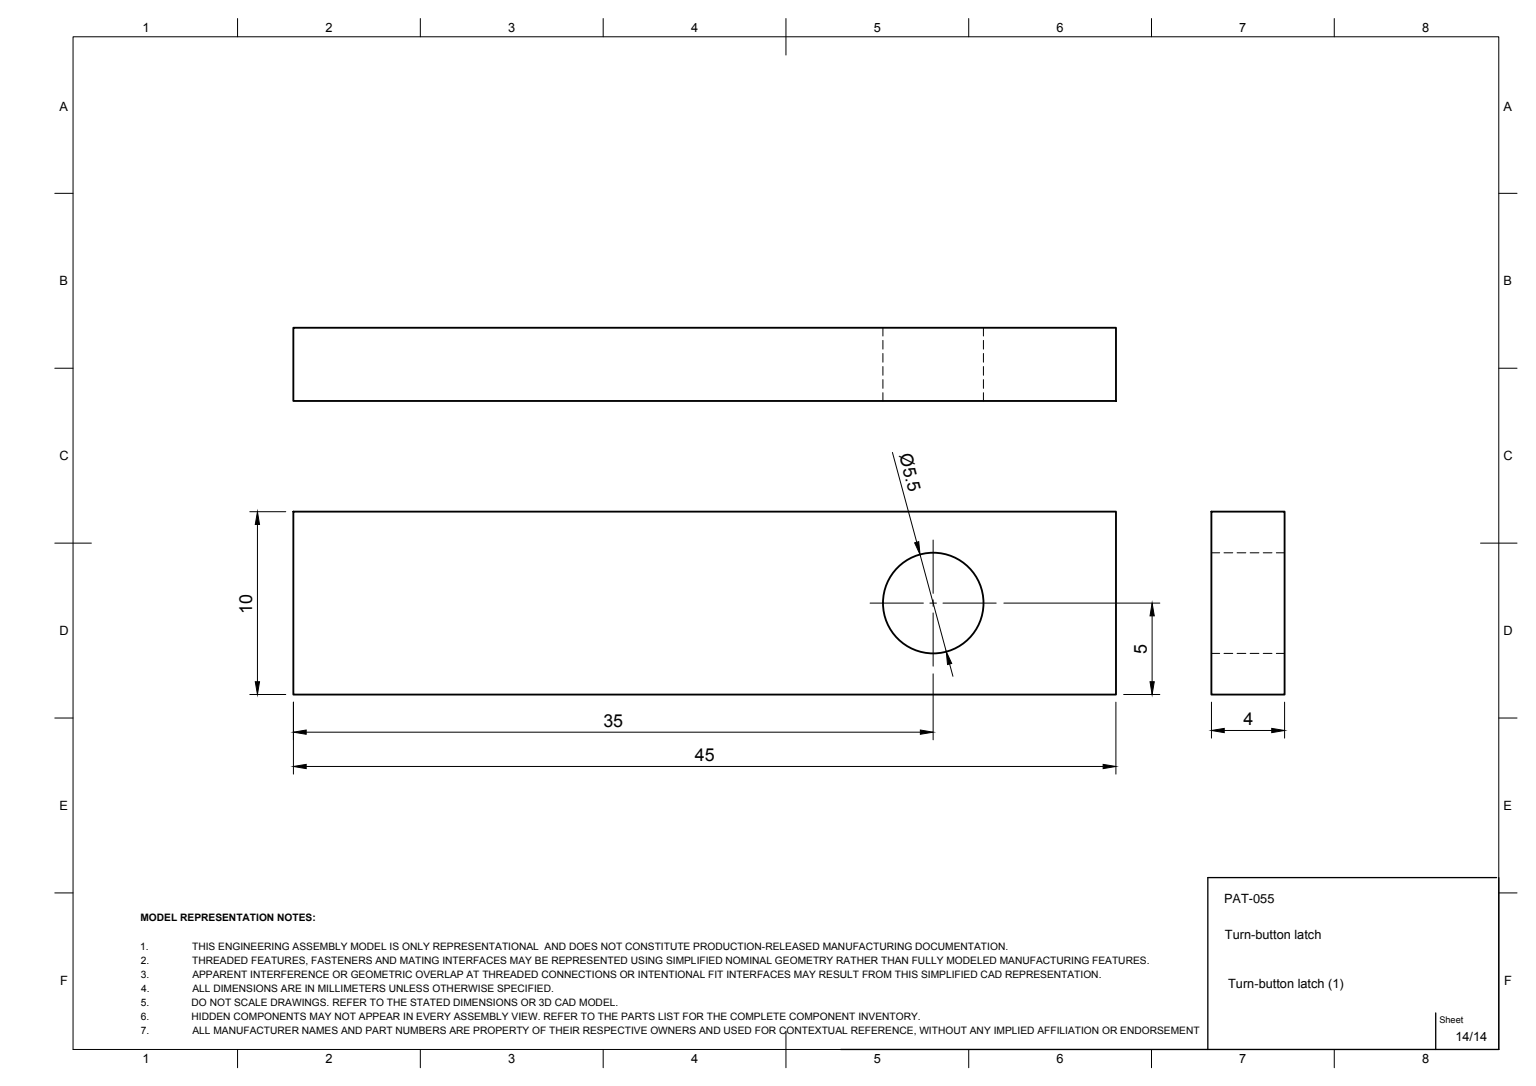
ISO-10303-21;
HEADER;
/* Generated by software containing ST-Developer
 * from STEP Tools, Inc. (www.steptools.com) 
 */

FILE_DESCRIPTION(
/* description */ ('Hinged panel with latch'),
/* implementation_level */ '2;1');

FILE_NAME(
/* name */ 'Turn-button latch (1).step',
/* time_stamp */ '2026-10-27T20:36:01-07:00',
/* author */ (''),
/* organization */ (''),
/* preprocessor_version */ 'ST-DEVELOPER v20.2',
/* originating_system */ 'Autodesk Translation Framework v15.17.0.0',
/* authorisation */ '');

FILE_SCHEMA (('AUTOMOTIVE_DESIGN { 1 0 10303 214 3 1 1 }'));
ENDSEC;

DATA;
#10=MECHANICAL_DESIGN_GEOMETRIC_PRESENTATION_REPRESENTATION('',(#311),#6743);
#279=SHAPE_REPRESENTATION_RELATIONSHIP('SRR','None',#6856,#295);
#295=ADVANCED_BREP_SHAPE_REPRESENTATION('',(#324),#6742);
#311=STYLED_ITEM('',(#6989),#324);
#324=MANIFOLD_SOLID_BREP('Body1',#3816);
#370=FACE_BOUND('',#975,.T.);
#371=FACE_BOUND('',#978,.T.);
#517=PLANE('',#4354);
#518=PLANE('',#4355);
#519=PLANE('',#4356);
#520=PLANE('',#4357);
#521=PLANE('',#4358);
#522=PLANE('',#4359);
#722=FACE_OUTER_BOUND('',#973,.T.);
#723=FACE_OUTER_BOUND('',#974,.T.);
#724=FACE_OUTER_BOUND('',#976,.T.);
#725=FACE_OUTER_BOUND('',#977,.T.);
#726=FACE_OUTER_BOUND('',#979,.T.);
#727=FACE_OUTER_BOUND('',#980,.T.);
#728=FACE_OUTER_BOUND('',#981,.T.);
#973=EDGE_LOOP('',(#3526,#3527,#3528,#3529));
#974=EDGE_LOOP('',(#3530,#3531,#3532,#3533));
#975=EDGE_LOOP('',(#3534));
#976=EDGE_LOOP('',(#3535,#3536,#3537,#3538));
#977=EDGE_LOOP('',(#3539,#3540,#3541,#3542));
#978=EDGE_LOOP('',(#3543));
#979=EDGE_LOOP('',(#3544,#3545,#3546,#3547));
#980=EDGE_LOOP('',(#3548,#3549,#3550,#3551));
#981=EDGE_LOOP('',(#3552,#3553,#3554,#3555));
#1327=LINE('',#6670,#1685);
#1328=LINE('',#6675,#1686);
#1329=LINE('',#6677,#1687);
#1330=LINE('',#6679,#1688);
#1331=LINE('',#6680,#1689);
#1332=LINE('',#6683,#1690);
#1333=LINE('',#6685,#1691);
#1334=LINE('',#6686,#1692);
#1335=LINE('',#6689,#1693);
#1336=LINE('',#6691,#1694);
#1337=LINE('',#6692,#1695);
#1338=LINE('',#6694,#1696);
#1339=LINE('',#6695,#1697);
#1685=VECTOR('',#5427,0.274999999999999);
#1686=VECTOR('',#5432,1.);
#1687=VECTOR('',#5433,1.);
#1688=VECTOR('',#5434,1.);
#1689=VECTOR('',#5435,1.);
#1690=VECTOR('',#5438,1.);
#1691=VECTOR('',#5439,1.);
#1692=VECTOR('',#5440,1.);
#1693=VECTOR('',#5443,1.);
#1694=VECTOR('',#5444,1.);
#1695=VECTOR('',#5445,1.);
#1696=VECTOR('',#5448,1.);
#1697=VECTOR('',#5449,1.);
#1789=CIRCLE('',#4352,0.274999999999999);
#1790=CIRCLE('',#4353,0.274999999999999);
#2097=VERTEX_POINT('',#6667);
#2098=VERTEX_POINT('',#6669);
#2099=VERTEX_POINT('',#6673);
#2100=VERTEX_POINT('',#6674);
#2101=VERTEX_POINT('',#6676);
#2102=VERTEX_POINT('',#6678);
#2103=VERTEX_POINT('',#6682);
#2104=VERTEX_POINT('',#6684);
#2105=VERTEX_POINT('',#6688);
#2106=VERTEX_POINT('',#6690);
#2575=EDGE_CURVE('',#2097,#2097,#1789,.T.);
#2576=EDGE_CURVE('',#2097,#2098,#1327,.T.);
#2577=EDGE_CURVE('',#2098,#2098,#1790,.T.);
#2578=EDGE_CURVE('',#2099,#2100,#1328,.T.);
#2579=EDGE_CURVE('',#2100,#2101,#1329,.T.);
#2580=EDGE_CURVE('',#2102,#2101,#1330,.T.);
#2581=EDGE_CURVE('',#2099,#2102,#1331,.T.);
#2582=EDGE_CURVE('',#2103,#2099,#1332,.T.);
#2583=EDGE_CURVE('',#2104,#2102,#1333,.T.);
#2584=EDGE_CURVE('',#2103,#2104,#1334,.T.);
#2585=EDGE_CURVE('',#2105,#2103,#1335,.T.);
#2586=EDGE_CURVE('',#2106,#2104,#1336,.T.);
#2587=EDGE_CURVE('',#2105,#2106,#1337,.T.);
#2588=EDGE_CURVE('',#2100,#2105,#1338,.T.);
#2589=EDGE_CURVE('',#2101,#2106,#1339,.T.);
#3526=ORIENTED_EDGE('',*,*,#2575,.F.);
#3527=ORIENTED_EDGE('',*,*,#2576,.T.);
#3528=ORIENTED_EDGE('',*,*,#2577,.F.);
#3529=ORIENTED_EDGE('',*,*,#2576,.F.);
#3530=ORIENTED_EDGE('',*,*,#2578,.T.);
#3531=ORIENTED_EDGE('',*,*,#2579,.T.);
#3532=ORIENTED_EDGE('',*,*,#2580,.F.);
#3533=ORIENTED_EDGE('',*,*,#2581,.F.);
#3534=ORIENTED_EDGE('',*,*,#2577,.T.);
#3535=ORIENTED_EDGE('',*,*,#2582,.T.);
#3536=ORIENTED_EDGE('',*,*,#2581,.T.);
#3537=ORIENTED_EDGE('',*,*,#2583,.F.);
#3538=ORIENTED_EDGE('',*,*,#2584,.F.);
#3539=ORIENTED_EDGE('',*,*,#2585,.T.);
#3540=ORIENTED_EDGE('',*,*,#2584,.T.);
#3541=ORIENTED_EDGE('',*,*,#2586,.F.);
#3542=ORIENTED_EDGE('',*,*,#2587,.F.);
#3543=ORIENTED_EDGE('',*,*,#2575,.T.);
#3544=ORIENTED_EDGE('',*,*,#2588,.T.);
#3545=ORIENTED_EDGE('',*,*,#2587,.T.);
#3546=ORIENTED_EDGE('',*,*,#2589,.F.);
#3547=ORIENTED_EDGE('',*,*,#2579,.F.);
#3548=ORIENTED_EDGE('',*,*,#2589,.T.);
#3549=ORIENTED_EDGE('',*,*,#2586,.T.);
#3550=ORIENTED_EDGE('',*,*,#2583,.T.);
#3551=ORIENTED_EDGE('',*,*,#2580,.T.);
#3552=ORIENTED_EDGE('',*,*,#2588,.F.);
#3553=ORIENTED_EDGE('',*,*,#2578,.F.);
#3554=ORIENTED_EDGE('',*,*,#2582,.F.);
#3555=ORIENTED_EDGE('',*,*,#2585,.F.);
#3591=CYLINDRICAL_SURFACE('',#4351,0.274999999999999);
#3791=ADVANCED_FACE('',(#722),#3591,.F.);
#3792=ADVANCED_FACE('',(#723,#370),#517,.T.);
#3793=ADVANCED_FACE('',(#724),#518,.T.);
#3794=ADVANCED_FACE('',(#725,#371),#519,.T.);
#3795=ADVANCED_FACE('',(#726),#520,.T.);
#3796=ADVANCED_FACE('',(#727),#521,.T.);
#3797=ADVANCED_FACE('',(#728),#522,.F.);
#3816=CLOSED_SHELL('',(#3791,#3792,#3793,#3794,#3795,#3796,#3797));
#4350=AXIS2_PLACEMENT_3D('',#6665,#5421,#5422);
#4351=AXIS2_PLACEMENT_3D('',#6666,#5423,#5424);
#4352=AXIS2_PLACEMENT_3D('',#6668,#5425,#5426);
#4353=AXIS2_PLACEMENT_3D('',#6671,#5428,#5429);
#4354=AXIS2_PLACEMENT_3D('',#6672,#5430,#5431);
#4355=AXIS2_PLACEMENT_3D('',#6681,#5436,#5437);
#4356=AXIS2_PLACEMENT_3D('',#6687,#5441,#5442);
#4357=AXIS2_PLACEMENT_3D('',#6693,#5446,#5447);
#4358=AXIS2_PLACEMENT_3D('',#6696,#5450,#5451);
#4359=AXIS2_PLACEMENT_3D('',#6697,#5452,#5453);
#5421=DIRECTION('axis',(0.,0.,1.));
#5422=DIRECTION('refdir',(1.,0.,0.));
#5423=DIRECTION('center_axis',(0.,1.,0.));
#5424=DIRECTION('ref_axis',(1.,0.,0.));
#5425=DIRECTION('center_axis',(0.,1.,0.));
#5426=DIRECTION('ref_axis',(1.,0.,0.));
#5427=DIRECTION('',(0.,1.,0.));
#5428=DIRECTION('center_axis',(0.,-1.,0.));
#5429=DIRECTION('ref_axis',(1.,0.,0.));
#5430=DIRECTION('center_axis',(0.,1.,0.));
#5431=DIRECTION('ref_axis',(-1.,0.,0.));
#5432=DIRECTION('',(-1.,0.,0.));
#5433=DIRECTION('',(0.,0.,1.));
#5434=DIRECTION('',(-1.,0.,0.));
#5435=DIRECTION('',(0.,0.,1.));
#5436=DIRECTION('center_axis',(1.,0.,0.));
#5437=DIRECTION('ref_axis',(0.,1.,0.));
#5438=DIRECTION('',(0.,1.,0.));
#5439=DIRECTION('',(0.,1.,0.));
#5440=DIRECTION('',(0.,0.,1.));
#5441=DIRECTION('center_axis',(0.,-1.,0.));
#5442=DIRECTION('ref_axis',(1.,0.,0.));
#5443=DIRECTION('',(1.,0.,0.));
#5444=DIRECTION('',(1.,0.,0.));
#5445=DIRECTION('',(0.,0.,1.));
#5446=DIRECTION('center_axis',(-1.,0.,0.));
#5447=DIRECTION('ref_axis',(0.,-1.,0.));
#5448=DIRECTION('',(0.,-1.,0.));
#5449=DIRECTION('',(0.,-1.,0.));
#5450=DIRECTION('center_axis',(0.,0.,1.));
#5451=DIRECTION('ref_axis',(1.,0.,0.));
#5452=DIRECTION('center_axis',(0.,0.,1.));
#5453=DIRECTION('ref_axis',(1.,0.,0.));
#6665=CARTESIAN_POINT('',(0.,0.,0.));
#6666=CARTESIAN_POINT('Origin',(20.,-2.3,16.));
#6667=CARTESIAN_POINT('',(19.725,-2.2,16.));
#6668=CARTESIAN_POINT('Origin',(20.,-2.2,16.));
#6669=CARTESIAN_POINT('',(19.725,-1.8,16.));
#6670=CARTESIAN_POINT('',(19.725,-2.3,16.));
#6671=CARTESIAN_POINT('Origin',(20.,-1.8,16.));
#6672=CARTESIAN_POINT('Origin',(23.5,-1.8,15.5));
#6673=CARTESIAN_POINT('',(23.5,-1.8,15.5));
#6674=CARTESIAN_POINT('',(19.,-1.8,15.5));
#6675=CARTESIAN_POINT('',(23.5,-1.8,15.5));
#6676=CARTESIAN_POINT('',(19.,-1.8,16.5));
#6677=CARTESIAN_POINT('',(19.,-1.8,15.5));
#6678=CARTESIAN_POINT('',(23.5,-1.8,16.5));
#6679=CARTESIAN_POINT('',(23.5,-1.8,16.5));
#6680=CARTESIAN_POINT('',(23.5,-1.8,15.5));
#6681=CARTESIAN_POINT('Origin',(23.5,-2.2,15.5));
#6682=CARTESIAN_POINT('',(23.5,-2.2,15.5));
#6683=CARTESIAN_POINT('',(23.5,-2.2,15.5));
#6684=CARTESIAN_POINT('',(23.5,-2.2,16.5));
#6685=CARTESIAN_POINT('',(23.5,-2.2,16.5));
#6686=CARTESIAN_POINT('',(23.5,-2.2,15.5));
#6687=CARTESIAN_POINT('Origin',(19.,-2.2,15.5));
#6688=CARTESIAN_POINT('',(19.,-2.2,15.5));
#6689=CARTESIAN_POINT('',(19.,-2.2,15.5));
#6690=CARTESIAN_POINT('',(19.,-2.2,16.5));
#6691=CARTESIAN_POINT('',(19.,-2.2,16.5));
#6692=CARTESIAN_POINT('',(19.,-2.2,15.5));
#6693=CARTESIAN_POINT('Origin',(19.,-1.8,15.5));
#6694=CARTESIAN_POINT('',(19.,-1.8,15.5));
#6695=CARTESIAN_POINT('',(19.,-1.8,16.5));
#6696=CARTESIAN_POINT('Origin',(21.25,-2.,16.5));
#6697=CARTESIAN_POINT('Origin',(21.25,-2.,15.5));
#6721=UNCERTAINTY_MEASURE_WITH_UNIT(LENGTH_MEASURE(0.001),#6744,
'DISTANCE_ACCURACY_VALUE',
'Maximum model space distance between geometric entities at asserted c
onnectivities');
#6722=UNCERTAINTY_MEASURE_WITH_UNIT(LENGTH_MEASURE(0.001),#6744,
'DISTANCE_ACCURACY_VALUE',
'Maximum model space distance between geometric entities at asserted c
onnectivities');
#6742=(
GEOMETRIC_REPRESENTATION_CONTEXT(3)
GLOBAL_UNCERTAINTY_ASSIGNED_CONTEXT((#6721))
GLOBAL_UNIT_ASSIGNED_CONTEXT((#6744,#6746,#6747))
REPRESENTATION_CONTEXT('','3D')
);
#6743=(
GEOMETRIC_REPRESENTATION_CONTEXT(3)
GLOBAL_UNCERTAINTY_ASSIGNED_CONTEXT((#6722))
GLOBAL_UNIT_ASSIGNED_CONTEXT((#6744,#6746,#6747))
REPRESENTATION_CONTEXT('','3D')
);
#6744=(
LENGTH_UNIT()
NAMED_UNIT(*)
SI_UNIT(.CENTI.,.METRE.)
);
#6746=(
NAMED_UNIT(*)
PLANE_ANGLE_UNIT()
SI_UNIT($,.RADIAN.)
);
#6747=(
NAMED_UNIT(*)
SI_UNIT($,.STERADIAN.)
SOLID_ANGLE_UNIT()
);
#6767=SHAPE_DEFINITION_REPRESENTATION(#6832,#6856);
#6832=PRODUCT_DEFINITION_SHAPE('',$,#6877);
#6856=SHAPE_REPRESENTATION('',(#4350),#6742);
#6857=PRODUCT_DEFINITION_CONTEXT('part definition',#6919,'design');
#6877=PRODUCT_DEFINITION('Turn-button latch (1)','Turn-button latch (1)',
#6897,#6857);
#6897=PRODUCT_DEFINITION_FORMATION('',$,#6940);
#6919=APPLICATION_CONTEXT(
'Core Data for Automotive Mechanical Design Process');
#6920=PRODUCT_CONTEXT('part definition',#6919,'mechanical');
#6940=PRODUCT('Turn-button latch (1)','Turn-button latch (1)',
'Turn-button latch (1)',(#6920));
#6983=COLOUR_RGB('Light Blue',0.38,0.62,0.78);
#6984=FILL_AREA_STYLE_COLOUR('',#6983);
#6985=FILL_AREA_STYLE('',(#6984));
#6986=SURFACE_STYLE_FILL_AREA(#6985);
#6987=SURFACE_SIDE_STYLE('',(#6986));
#6988=SURFACE_STYLE_USAGE(.BOTH.,#6987);
#6989=PRESENTATION_STYLE_ASSIGNMENT((#6988));
ENDSEC;
END-ISO-10303-21;
